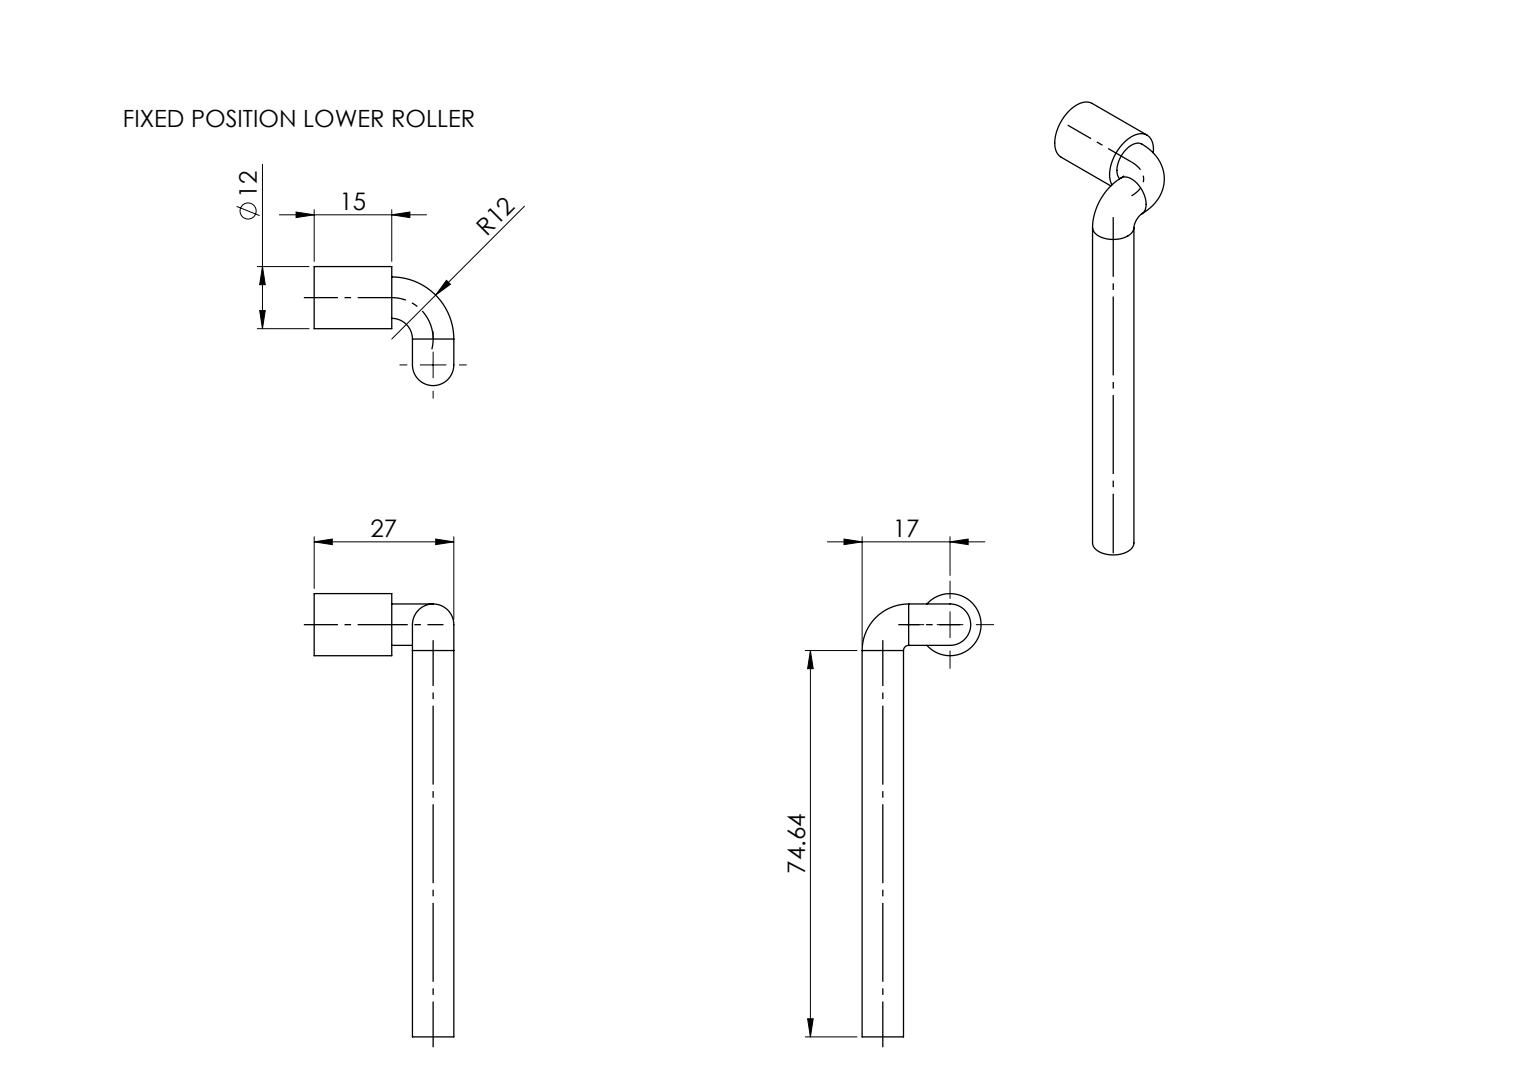
ISO-10303-21;
HEADER;
FILE_DESCRIPTION (('STEP AP214'),
    '1' );
FILE_NAME ('fixed position lower roller.step',
    '2026-10-03T20:08:58',
    ( '' ),
    ( '' ),
    'SwSTEP 2.0',
    'SolidWorks 2026',
    '' );
FILE_SCHEMA (( 'AUTOMOTIVE_DESIGN' ));
ENDSEC;

DATA;
#39=SHAPE_DEFINITION_REPRESENTATION ( #2484, #8378 ) ;
#44=PLANE ( 'NONE',  #3777 ) ;
#107=CIRCLE ( 'NONE', #5659, 4.000000000000001776 ) ;
#165=CARTESIAN_POINT ( 'NONE',  ( 14.00000000000000000, -30.00000000000000000, 0.000000000000000000 ) ) ;
#183=EDGE_CURVE ( 'NONE', #1508, #4176, #5201, .T. ) ;
#196=AXIS2_PLACEMENT_3D ( 'NONE', #1167, #8956, #10887 ) ;
#219=ORIENTED_EDGE ( 'NONE', *, *, #11430, .T. ) ;
#239=CIRCLE ( 'NONE', #9478, 4.000000000000001776 ) ;
#289=DIRECTION ( 'NONE',  ( 0.000000000000000000, 0.000000000000000000, 1.000000000000000000 ) ) ;
#309=CARTESIAN_POINT ( 'NONE',  ( 14.00000000000000000, 45.63999999999998636, -5.000000000000001776 ) ) ;
#315=DIRECTION ( 'NONE',  ( 0.000000000000000000, -1.000000000000000000, 0.000000000000000000 ) ) ;
#335=VERTEX_POINT ( 'NONE', #4396 ) ;
#383=CIRCLE ( 'NONE', #8612, 3.999999999999997335 ) ;
#411=DIRECTION ( 'NONE',  ( 1.000000000000000000, -0.000000000000000000, -0.000000000000000000 ) ) ;
#441=DIRECTION ( 'NONE',  ( 1.000000000000000000, 0.000000000000000000, 0.000000000000000000 ) ) ;
#461=( NAMED_UNIT ( * ) SI_UNIT ( $, .STERADIAN. ) SOLID_ANGLE_UNIT ( ) );
#467=DIRECTION ( 'NONE',  ( 0.000000000000000000, 0.000000000000000000, -1.000000000000000000 ) ) ;
#526=FILL_AREA_STYLE ('',( #12323 ) ) ;
#598=COLOUR_RGB ( '', 0.40784314, 0.44705882, 0.49803922) ;
#623=CIRCLE ( 'NONE', #8615, 4.000000000000001776 ) ;
#633=TOROIDAL_SURFACE ( 'NONE', #12373, 4.999999999999997335, 4.000000000000000000 ) ;
#644=AXIS2_PLACEMENT_3D ( 'NONE', #4663, #8717, #5810 ) ;
#663=EDGE_CURVE ( 'NONE', #8684, #9579, #239, .T. ) ;
#710=CIRCLE ( 'NONE', #1557, 12.00000000000000000 ) ;
#712=AXIS2_PLACEMENT_3D ( 'NONE', #10541, #1663, #1727 ) ;
#726=ADVANCED_FACE ( 'NONE', ( #8496 ), #11276, .T. ) ;
#750=DIRECTION ( 'NONE',  ( 0.000000000000000000, -1.000000000000000000, 0.000000000000000000 ) ) ;
#801=FACE_OUTER_BOUND ( 'NONE', #953, .T. ) ;
#853=CARTESIAN_POINT ( 'NONE',  ( 6.000000000000000000, 49.63999999999998636, -5.000000000000000888 ) ) ;
#868=ORIENTED_EDGE ( 'NONE', *, *, #10999, .F. ) ;
#953=EDGE_LOOP ( 'NONE', ( #2112, #9197, #11094, #219, #1705 ) ) ;
#990=ORIENTED_EDGE ( 'NONE', *, *, #11430, .F. ) ;
#1013=( GEOMETRIC_REPRESENTATION_CONTEXT ( 3 ) GLOBAL_UNCERTAINTY_ASSIGNED_CONTEXT ( ( #8516 ) ) GLOBAL_UNIT_ASSIGNED_CONTEXT ( ( #5432, #1437, #12211 ) ) REPRESENTATION_CONTEXT ( 'NONE', 'WORKASPACE' ) );
#1035=COLOUR_RGB ( '', 0.40784314, 0.44705882, 0.49803922) ;
#1075=EDGE_CURVE ( 'NONE', #9359, #4176, #10389, .T. ) ;
#1167=CARTESIAN_POINT ( 'NONE',  ( 6.000000000000000000, 49.63999999999998636, -13.00000000000000178 ) ) ;
#1182=VERTEX_POINT ( 'NONE', #6546 ) ;
#1304=CARTESIAN_POINT ( 'NONE',  ( 18.00000000000000355, 49.63999999999998636, -5.000000000000002665 ) ) ;
#1317=DIRECTION ( 'NONE',  ( 0.000000000000000000, -0.000000000000000000, -1.000000000000000000 ) ) ;
#1361=ORIENTED_EDGE ( 'NONE', *, *, #8700, .T. ) ;
#1370=EDGE_CURVE ( 'NONE', #1182, #3532, #383, .T. ) ;
#1431=PLANE ( 'NONE',  #6524 ) ;
#1437=( NAMED_UNIT ( * ) PLANE_ANGLE_UNIT ( ) SI_UNIT ( $, .RADIAN. ) );
#1456=DIRECTION ( 'NONE',  ( 0.000000000000000000, 0.000000000000000000, -1.000000000000000000 ) ) ;
#1467=CARTESIAN_POINT ( 'NONE',  ( -9.000000000000000000, 49.63999999999998636, -7.000000000000000888 ) ) ;
#1477=EDGE_CURVE ( 'NONE', #4665, #9359, #3885, .T. ) ;
#1508=VERTEX_POINT ( 'NONE', #12741 ) ;
#1527=CARTESIAN_POINT ( 'NONE',  ( 14.00000000000000000, -30.00000000000000000, 0.000000000000000000 ) ) ;
#1554=( NAMED_UNIT ( * ) PLANE_ANGLE_UNIT ( ) SI_UNIT ( $, .RADIAN. ) );
#1557=AXIS2_PLACEMENT_3D ( 'NONE', #2137, #6252, #4257 ) ;
#1576=DIRECTION ( 'NONE',  ( 0.000000000000000000, -1.000000000000000000, 0.000000000000000000 ) ) ;
#1583=DIRECTION ( 'NONE',  ( -1.000000000000000000, 0.000000000000000000, 0.000000000000000000 ) ) ;
#1615=SHAPE_REPRESENTATION_RELATIONSHIP ( 'NONE' , 'NONE' ,  #8378, #2668 ) ;
#1663=DIRECTION ( 'NONE',  ( 1.000000000000000000, -0.000000000000000000, -0.000000000000000000 ) ) ;
#1667=ADVANCED_FACE ( 'NONE', ( #7835 ), #4159, .T. ) ;
#1687=DIRECTION ( 'NONE',  ( 0.000000000000000000, 0.000000000000000000, 1.000000000000000000 ) ) ;
#1705=ORIENTED_EDGE ( 'NONE', *, *, #9638, .F. ) ;
#1721=DIRECTION ( 'NONE',  ( 0.000000000000000000, 0.000000000000000000, 1.000000000000000000 ) ) ;
#1727=DIRECTION ( 'NONE',  ( 0.000000000000000000, 0.000000000000000000, -1.000000000000000000 ) ) ;
#1775=ORIENTED_EDGE ( 'NONE', *, *, #8895, .T. ) ;
#1784=ORIENTED_EDGE ( 'NONE', *, *, #6220, .F. ) ;
#1797=ORIENTED_EDGE ( 'NONE', *, *, #2499, .F. ) ;
#1867=EDGE_LOOP ( 'NONE', ( #3480, #9604, #3827, #3918 ) ) ;
#2007=FACE_BOUND ( 'NONE', #4689, .T. ) ;
#2111=ORIENTED_EDGE ( 'NONE', *, *, #4710, .T. ) ;
#2112=ORIENTED_EDGE ( 'NONE', *, *, #6635, .F. ) ;
#2137=CARTESIAN_POINT ( 'NONE',  ( 6.000000000000000000, 49.63999999999998636, -5.000000000000000888 ) ) ;
#2180=ORIENTED_EDGE ( 'NONE', *, *, #9546, .F. ) ;
#2213=CARTESIAN_POINT ( 'NONE',  ( 6.000000000000000000, 49.63999999999998636, -13.00000000000000178 ) ) ;
#2355=SURFACE_STYLE_USAGE ( .BOTH. , #11170 ) ;
#2484=PRODUCT_DEFINITION_SHAPE ( 'NONE', 'NONE',  #5392 ) ;
#2492=EDGE_LOOP ( 'NONE', ( #5472, #2661, #6374, #990, #2581 ) ) ;
#2499=EDGE_CURVE ( 'NONE', #6983, #335, #11734, .T. ) ;
#2512=CARTESIAN_POINT ( 'NONE',  ( 14.00000000000000000, 49.63999999999998636, -5.000000000000001776 ) ) ;
#2540=CARTESIAN_POINT ( 'NONE',  ( -9.000000000000000000, 49.63999999999998636, -13.00000000000000178 ) ) ;
#2543=CARTESIAN_POINT ( 'NONE',  ( 14.00000000000000000, 61.31370849898475228, 3.999999999999997335 ) ) ;
#2565=ORIENTED_EDGE ( 'NONE', *, *, #663, .F. ) ;
#2581=ORIENTED_EDGE ( 'NONE', *, *, #4127, .T. ) ;
#2596=SURFACE_SIDE_STYLE ('',( #11353 ) ) ;
#2657=CARTESIAN_POINT ( 'NONE',  ( 14.00000000000000000, 49.63999999999998636, -5.000000000000001776 ) ) ;
#2661=ORIENTED_EDGE ( 'NONE', *, *, #6635, .T. ) ;
#2668=ADVANCED_BREP_SHAPE_REPRESENTATION ( '', ( #10172, #12422 ), #7225 ) ;
#2717=MECHANICAL_DESIGN_GEOMETRIC_PRESENTATION_REPRESENTATION('',(#4122),#5979);
#2801=AXIS2_PLACEMENT_3D ( 'NONE', #10218, #9264, #3434 ) ;
#2832=VERTEX_POINT ( 'NONE', #309 ) ;
#2874=DIRECTION ( 'NONE',  ( -0.000000000000000000, -1.000000000000000000, 0.000000000000000000 ) ) ;
#2906=APPLICATION_CONTEXT ( 'automotive_design' ) ;
#2926=ORIENTED_EDGE ( 'NONE', *, *, #1477, .F. ) ;
#3002=TOROIDAL_SURFACE ( 'NONE', #5451, 8.000000000000000000, 4.000000000000000000 ) ;
#3030=DIRECTION ( 'NONE',  ( 1.084202172485504434E-16, 0.000000000000000000, 1.000000000000000000 ) ) ;
#3084=DIRECTION ( 'NONE',  ( 0.000000000000000000, -1.000000000000000000, 0.000000000000000000 ) ) ;
#3123=ADVANCED_FACE ( 'NONE', ( #4941 ), #44, .T. ) ;
#3186=CYLINDRICAL_SURFACE ( 'NONE', #4205, 3.999999999999997335 ) ;
#3333=EDGE_LOOP ( 'NONE', ( #4773, #7781 ) ) ;
#3345=ORIENTED_EDGE ( 'NONE', *, *, #183, .F. ) ;
#3434=DIRECTION ( 'NONE',  ( 0.000000000000000000, 0.000000000000000000, 1.000000000000000000 ) ) ;
#3452=CARTESIAN_POINT ( 'NONE',  ( 14.00000000000000000, -30.00000000000000000, 0.000000000000000000 ) ) ;
#3480=ORIENTED_EDGE ( 'NONE', *, *, #7586, .T. ) ;
#3509=DIRECTION ( 'NONE',  ( 0.000000000000000000, -1.000000000000000000, 0.000000000000000000 ) ) ;
#3532=VERTEX_POINT ( 'NONE', #7691 ) ;
#3649=CARTESIAN_POINT ( 'NONE',  ( 14.00000000000000000, 61.31370849898475228, -3.999999999999997335 ) ) ;
#3777=AXIS2_PLACEMENT_3D ( 'NONE', #165, #3084, #1317 ) ;
#3801=CIRCLE ( 'NONE', #12246, 4.000000000000000000 ) ;
#3827=ORIENTED_EDGE ( 'NONE', *, *, #1370, .F. ) ;
#3856=PRODUCT_DEFINITION_FORMATION_WITH_SPECIFIED_SOURCE ( 'ANY', '', #11216, .NOT_KNOWN. ) ;
#3869=CARTESIAN_POINT ( 'NONE',  ( 6.000000000000000000, 49.63999999999998636, -5.000000000000000888 ) ) ;
#3885=CIRCLE ( 'NONE', #9832, 6.000000000000000000 ) ;
#3918=ORIENTED_EDGE ( 'NONE', *, *, #4710, .F. ) ;
#4087=ORIENTED_EDGE ( 'NONE', *, *, #7899, .F. ) ;
#4097=ORIENTED_EDGE ( 'NONE', *, *, #9546, .T. ) ;
#4122=STYLED_ITEM ( 'NONE', ( #5487 ), #2668 ) ;
#4127=EDGE_CURVE ( 'NONE', #2832, #8684, #4814, .T. ) ;
#4159=CYLINDRICAL_SURFACE ( 'NONE', #11300, 6.000000000000000000 ) ;
#4176=VERTEX_POINT ( 'NONE', #1467 ) ;
#4205=AXIS2_PLACEMENT_3D ( 'NONE', #9971, #11021, #9081 ) ;
#4257=DIRECTION ( 'NONE',  ( 0.000000000000000000, 0.000000000000000000, -1.000000000000000000 ) ) ;
#4314=AXIS2_PLACEMENT_3D ( 'NONE', #6303, #6240, #12180 ) ;
#4340=FILL_AREA_STYLE_COLOUR ( '', #598 ) ;
#4396=CARTESIAN_POINT ( 'NONE',  ( 6.000000000000000000, 49.63999999999998636, -17.00000000000000000 ) ) ;
#4457=( LENGTH_UNIT ( ) NAMED_UNIT ( * ) SI_UNIT ( .MILLI., .METRE. ) );
#4593=DIRECTION ( 'NONE',  ( -1.000000000000000000, 0.000000000000000000, 0.000000000000000000 ) ) ;
#4599=DIRECTION ( 'NONE',  ( 1.000000000000000000, 0.000000000000000000, 0.000000000000000000 ) ) ;
#4601=LINE ( 'NONE', #8514, #11819 ) ;
#4611=LINE ( 'NONE', #3649, #8149 ) ;
#4663=CARTESIAN_POINT ( 'NONE',  ( 14.00000000000000000, 44.64000000000000057, -5.000000000000000888 ) ) ;
#4665=VERTEX_POINT ( 'NONE', #12412 ) ;
#4689=EDGE_LOOP ( 'NONE', ( #1797, #11902 ) ) ;
#4710=EDGE_CURVE ( 'NONE', #9185, #1182, #4611, .T. ) ;
#4733=CIRCLE ( 'NONE', #4314, 6.000000000000000000 ) ;
#4735=DIRECTION ( 'NONE',  ( -1.000000000000000000, 0.000000000000000000, 0.000000000000000000 ) ) ;
#4773=ORIENTED_EDGE ( 'NONE', *, *, #10875, .T. ) ;
#4814=CIRCLE ( 'NONE', #10984, 4.000000000000001776 ) ;
#4941=FACE_OUTER_BOUND ( 'NONE', #6769, .T. ) ;
#4961=DIRECTION ( 'NONE',  ( 0.000000000000000000, 0.000000000000000000, -1.000000000000000000 ) ) ;
#5078=ADVANCED_FACE ( 'NONE', ( #6464 ), #1431, .F. ) ;
#5201=CIRCLE ( 'NONE', #7672, 6.000000000000000000 ) ;
#5365=DIRECTION ( 'NONE',  ( 0.000000000000000000, 0.000000000000000000, -1.000000000000000000 ) ) ;
#5382=CIRCLE ( 'NONE', #12189, 4.000000000000000000 ) ;
#5384=ORIENTED_EDGE ( 'NONE', *, *, #8895, .F. ) ;
#5392=PRODUCT_DEFINITION ( 'UNKNOWN', '', #3856, #11070 ) ;
#5429=CIRCLE ( 'NONE', #11614, 3.999999999999997335 ) ;
#5432=( LENGTH_UNIT ( ) NAMED_UNIT ( * ) SI_UNIT ( .MILLI., .METRE. ) );
#5451=AXIS2_PLACEMENT_3D ( 'NONE', #3869, #5728, #4961 ) ;
#5472=ORIENTED_EDGE ( 'NONE', *, *, #663, .T. ) ;
#5487=PRESENTATION_STYLE_ASSIGNMENT (( #10435 ) ) ;
#5503=FACE_OUTER_BOUND ( 'NONE', #2492, .T. ) ;
#5506=ORIENTED_EDGE ( 'NONE', *, *, #2499, .T. ) ;
#5566=FACE_OUTER_BOUND ( 'NONE', #9035, .T. ) ;
#5596=ORIENTED_EDGE ( 'NONE', *, *, #6633, .F. ) ;
#5659=AXIS2_PLACEMENT_3D ( 'NONE', #7893, #3030, #10920 ) ;
#5706=ORIENTED_EDGE ( 'NONE', *, *, #8700, .F. ) ;
#5707=CARTESIAN_POINT ( 'NONE',  ( 0.000000000000000000, 0.000000000000000000, 0.000000000000000000 ) ) ;
#5728=DIRECTION ( 'NONE',  ( -0.000000000000000000, -1.000000000000000000, 0.000000000000000000 ) ) ;
#5754=AXIS2_PLACEMENT_3D ( 'NONE', #6221, #10326, #1456 ) ;
#5774=DIRECTION ( 'NONE',  ( -0.000000000000000000, -1.000000000000000000, 0.000000000000000000 ) ) ;
#5810=DIRECTION ( 'NONE',  ( 0.000000000000000000, 0.000000000000000000, -1.000000000000000000 ) ) ;
#5825=DIRECTION ( 'NONE',  ( 0.000000000000000000, 0.000000000000000000, -1.000000000000000000 ) ) ;
#5953=ORIENTED_EDGE ( 'NONE', *, *, #1477, .T. ) ;
#5979=( GEOMETRIC_REPRESENTATION_CONTEXT ( 3 ) GLOBAL_UNCERTAINTY_ASSIGNED_CONTEXT ( ( #10346 ) ) GLOBAL_UNIT_ASSIGNED_CONTEXT ( ( #11284, #8444, #461 ) ) REPRESENTATION_CONTEXT ( 'NONE', 'WORKASPACE' ) );
#6059=FACE_OUTER_BOUND ( 'NONE', #12004, .T. ) ;
#6106=ORIENTED_EDGE ( 'NONE', *, *, #11647, .T. ) ;
#6130=DIRECTION ( 'NONE',  ( 0.000000000000000000, 0.000000000000000000, 1.000000000000000000 ) ) ;
#6140=DIRECTION ( 'NONE',  ( 0.000000000000000000, -1.000000000000000000, 0.000000000000000000 ) ) ;
#6173=AXIS2_PLACEMENT_3D ( 'NONE', #9380, #8432, #11275 ) ;
#6195=CIRCLE ( 'NONE', #644, 0.9999999999999974465 ) ;
#6220=EDGE_CURVE ( 'NONE', #11818, #3532, #12396, .T. ) ;
#6221=CARTESIAN_POINT ( 'NONE',  ( 14.00000000000000000, 61.31370849898475228, 0.000000000000000000 ) ) ;
#6240=DIRECTION ( 'NONE',  ( -1.000000000000000000, 0.000000000000000000, 0.000000000000000000 ) ) ;
#6252=DIRECTION ( 'NONE',  ( -0.000000000000000000, -1.000000000000000000, 0.000000000000000000 ) ) ;
#6288=FACE_OUTER_BOUND ( 'NONE', #1867, .T. ) ;
#6303=CARTESIAN_POINT ( 'NONE',  ( 6.000000000000000000, 49.63999999999998636, -13.00000000000000178 ) ) ;
#6367=STYLED_ITEM ( 'NONE', ( #11365 ), #10172 ) ;
#6374=ORIENTED_EDGE ( 'NONE', *, *, #7586, .F. ) ;
#6398=CARTESIAN_POINT ( 'NONE',  ( -9.000000000000000000, 49.63999999999998636, -13.00000000000000178 ) ) ;
#6423=ORIENTED_EDGE ( 'NONE', *, *, #1370, .T. ) ;
#6425=CARTESIAN_POINT ( 'NONE',  ( -9.000000000000000000, 49.63999999999998636, -13.00000000000000178 ) ) ;
#6428=DIRECTION ( 'NONE',  ( 1.000000000000000000, 0.000000000000000000, 0.000000000000000000 ) ) ;
#6464=FACE_OUTER_BOUND ( 'NONE', #3333, .T. ) ;
#6501=DIRECTION ( 'NONE',  ( 1.084202172485504434E-16, 0.000000000000000000, 1.000000000000000000 ) ) ;
#6524=AXIS2_PLACEMENT_3D ( 'NONE', #6398, #10233, #467 ) ;
#6546=CARTESIAN_POINT ( 'NONE',  ( 14.00000000000000000, -30.00000000000000000, -3.999999999999997335 ) ) ;
#6598=AXIS2_PLACEMENT_3D ( 'NONE', #6425, #1583, #12053 ) ;
#6633=EDGE_CURVE ( 'NONE', #6983, #8089, #3801, .T. ) ;
#6635=EDGE_CURVE ( 'NONE', #9579, #11818, #11832, .T. ) ;
#6682=DIRECTION ( 'NONE',  ( 1.084202172485504434E-16, 0.000000000000000000, 1.000000000000000000 ) ) ;
#6696=CARTESIAN_POINT ( 'NONE',  ( 6.000000000000000000, 49.63999999999998636, -5.000000000000000888 ) ) ;
#6698=ORIENTED_EDGE ( 'NONE', *, *, #10875, .F. ) ;
#6767=CARTESIAN_POINT ( 'NONE',  ( 10.00000000000000000, 49.63999999999998636, -5.000000000000000888 ) ) ;
#6769=EDGE_LOOP ( 'NONE', ( #6423, #1361 ) ) ;
#6846=EDGE_CURVE ( 'NONE', #8089, #2832, #107, .T. ) ;
#6870=EDGE_LOOP ( 'NONE', ( #5384, #5953, #11441, #3345 ) ) ;
#6941=VECTOR ( 'NONE', #12458, 1000.000000000000000 ) ;
#6983=VERTEX_POINT ( 'NONE', #12097 ) ;
#7125=DIRECTION ( 'NONE',  ( -1.000000000000000000, 0.000000000000000000, 0.000000000000000000 ) ) ;
#7225=( GEOMETRIC_REPRESENTATION_CONTEXT ( 3 ) GLOBAL_UNCERTAINTY_ASSIGNED_CONTEXT ( ( #9438 ) ) GLOBAL_UNIT_ASSIGNED_CONTEXT ( ( #4457, #1554, #9150 ) ) REPRESENTATION_CONTEXT ( 'NONE', 'WORKASPACE' ) );
#7249=AXIS2_PLACEMENT_3D ( 'NONE', #853, #2874, #11681 ) ;
#7371=SURFACE_STYLE_FILL_AREA ( #10239 ) ;
#7392=DIRECTION ( 'NONE',  ( 0.000000000000000000, 0.000000000000000000, 1.000000000000000000 ) ) ;
#7434=DIRECTION ( 'NONE',  ( -1.000000000000000000, 0.000000000000000000, 0.000000000000000000 ) ) ;
#7586=EDGE_CURVE ( 'NONE', #9185, #11818, #8122, .T. ) ;
#7664=CLOSED_SHELL ( 'NONE', ( #11318, #8093, #726, #9848, #3123, #7850, #9969, #11541, #1667, #10336, #5078 ) ) ;
#7672=AXIS2_PLACEMENT_3D ( 'NONE', #2540, #4593, #1687 ) ;
#7691=CARTESIAN_POINT ( 'NONE',  ( 14.00000000000000000, -30.00000000000000000, 3.999999999999997335 ) ) ;
#7781=ORIENTED_EDGE ( 'NONE', *, *, #183, .T. ) ;
#7829=DIRECTION ( 'NONE',  ( 1.000000000000000000, 0.000000000000000000, -2.168404344971007882E-16 ) ) ;
#7835=FACE_OUTER_BOUND ( 'NONE', #6870, .T. ) ;
#7850=ADVANCED_FACE ( 'NONE', ( #6059 ), #3186, .T. ) ;
#7869=PLANE ( 'NONE',  #196 ) ;
#7893=CARTESIAN_POINT ( 'NONE',  ( 14.00000000000000000, 49.63999999999998636, -5.000000000000001776 ) ) ;
#7899=EDGE_CURVE ( 'NONE', #335, #8684, #710, .T. ) ;
#8067=EDGE_LOOP ( 'NONE', ( #2180, #2926 ) ) ;
#8072=PRODUCT_CONTEXT ( 'NONE', #12271, 'mechanical' ) ;
#8089=VERTEX_POINT ( 'NONE', #6767 ) ;
#8093=ADVANCED_FACE ( 'NONE', ( #8695 ), #3002, .T. ) ;
#8101=CARTESIAN_POINT ( 'NONE',  ( 14.00000000000000000, 53.63999999999999346, -5.000000000000001776 ) ) ;
#8122=CIRCLE ( 'NONE', #12055, 4.000000000000001776 ) ;
#8149=VECTOR ( 'NONE', #1576, 1000.000000000000000 ) ;
#8174=CARTESIAN_POINT ( 'NONE',  ( 14.00000000000000000, 44.64000000000000057, -6.938893903907228378E-15 ) ) ;
#8253=CARTESIAN_POINT ( 'NONE',  ( 14.00000000000000000, 44.64000000000000057, -4.000000000000007105 ) ) ;
#8265=TOROIDAL_SURFACE ( 'NONE', #7249, 8.000000000000000000, 4.000000000000000000 ) ;
#8378=SHAPE_REPRESENTATION ( 'fixed position lower roller', ( #12422 ), #7225 ) ;
#8432=DIRECTION ( 'NONE',  ( 1.000000000000000000, -0.000000000000000000, -0.000000000000000000 ) ) ;
#8444=( NAMED_UNIT ( * ) PLANE_ANGLE_UNIT ( ) SI_UNIT ( $, .RADIAN. ) );
#8496=FACE_OUTER_BOUND ( 'NONE', #12428, .T. ) ;
#8499=CARTESIAN_POINT ( 'NONE',  ( 6.000000000000000000, 49.63999999999998636, -7.000000000000000888 ) ) ;
#8514=CARTESIAN_POINT ( 'NONE',  ( 6.000000000000000000, 49.63999999999998636, -19.00000000000000355 ) ) ;
#8516=UNCERTAINTY_MEASURE_WITH_UNIT (LENGTH_MEASURE( 1.000000000000000082E-05 ), #5432, 'distance_accuracy_value', 'NONE');
#8591=CARTESIAN_POINT ( 'NONE',  ( 6.000000000000000000, 49.63999999999998636, -7.000000000000000888 ) ) ;
#8612=AXIS2_PLACEMENT_3D ( 'NONE', #1527, #750, #10598 ) ;
#8615=AXIS2_PLACEMENT_3D ( 'NONE', #9610, #6682, #7829 ) ;
#8629=VECTOR ( 'NONE', #4735, 1000.000000000000000 ) ;
#8684=VERTEX_POINT ( 'NONE', #1304 ) ;
#8695=FACE_OUTER_BOUND ( 'NONE', #11687, .T. ) ;
#8700=EDGE_CURVE ( 'NONE', #3532, #1182, #5429, .T. ) ;
#8717=DIRECTION ( 'NONE',  ( 1.000000000000000000, -0.000000000000000000, -0.000000000000000000 ) ) ;
#8857=ORIENTED_EDGE ( 'NONE', *, *, #4127, .F. ) ;
#8895=EDGE_CURVE ( 'NONE', #4665, #1508, #4601, .T. ) ;
#8956=DIRECTION ( 'NONE',  ( -1.000000000000000000, 0.000000000000000000, 0.000000000000000000 ) ) ;
#9035=EDGE_LOOP ( 'NONE', ( #4087, #6106, #9609, #868, #2565 ) ) ;
#9045=CARTESIAN_POINT ( 'NONE',  ( 6.000000000000000000, 49.63999999999998636, -13.00000000000000178 ) ) ;
#9081=DIRECTION ( 'NONE',  ( 0.000000000000000000, 0.000000000000000000, -1.000000000000000000 ) ) ;
#9150=( NAMED_UNIT ( * ) SI_UNIT ( $, .STERADIAN. ) SOLID_ANGLE_UNIT ( ) );
#9185=VERTEX_POINT ( 'NONE', #8253 ) ;
#9197=ORIENTED_EDGE ( 'NONE', *, *, #10999, .T. ) ;
#9264=DIRECTION ( 'NONE',  ( -1.000000000000000000, 0.000000000000000000, 0.000000000000000000 ) ) ;
#9268=TOROIDAL_SURFACE ( 'NONE', #12182, 4.999999999999997335, 4.000000000000000000 ) ;
#9359=VERTEX_POINT ( 'NONE', #8499 ) ;
#9380=CARTESIAN_POINT ( 'NONE',  ( 6.000000000000000000, 49.63999999999998636, -13.00000000000000178 ) ) ;
#9404=CARTESIAN_POINT ( 'NONE',  ( 14.00000000000000000, 44.64000000000000057, -5.000000000000000888 ) ) ;
#9437=CIRCLE ( 'NONE', #11721, 4.000000000000001776 ) ;
#9438=UNCERTAINTY_MEASURE_WITH_UNIT (LENGTH_MEASURE( 1.000000000000000082E-05 ), #4457, 'distance_accuracy_value', 'NONE');
#9467=CARTESIAN_POINT ( 'NONE',  ( 14.00000000000000000, 44.64000000000000057, -6.938893903907228378E-15 ) ) ;
#9478=AXIS2_PLACEMENT_3D ( 'NONE', #2657, #11344, #10426 ) ;
#9546=EDGE_CURVE ( 'NONE', #9359, #4665, #4733, .T. ) ;
#9563=DIRECTION ( 'NONE',  ( 0.000000000000000000, 0.000000000000000000, -1.000000000000000000 ) ) ;
#9579=VERTEX_POINT ( 'NONE', #8101 ) ;
#9604=ORIENTED_EDGE ( 'NONE', *, *, #6220, .T. ) ;
#9609=ORIENTED_EDGE ( 'NONE', *, *, #6633, .T. ) ;
#9610=CARTESIAN_POINT ( 'NONE',  ( 14.00000000000000000, 49.63999999999998636, -5.000000000000001776 ) ) ;
#9619=CARTESIAN_POINT ( 'NONE',  ( 6.000000000000000000, 49.63999999999998636, -13.00000000000000178 ) ) ;
#9638=EDGE_CURVE ( 'NONE', #11818, #9185, #9437, .T. ) ;
#9832=AXIS2_PLACEMENT_3D ( 'NONE', #9619, #12617, #1721 ) ;
#9848=ADVANCED_FACE ( 'NONE', ( #6288 ), #10261, .T. ) ;
#9969=ADVANCED_FACE ( 'NONE', ( #801 ), #633, .T. ) ;
#9971=CARTESIAN_POINT ( 'NONE',  ( 14.00000000000000000, 61.31370849898475228, 0.000000000000000000 ) ) ;
#9975=DIRECTION ( 'NONE',  ( 1.000000000000000000, -0.000000000000000000, -0.000000000000000000 ) ) ;
#10172=MANIFOLD_SOLID_BREP ( 'Boss-Extrude2', #7664 ) ;
#10218=CARTESIAN_POINT ( 'NONE',  ( 6.000000000000000000, 49.63999999999998636, -13.00000000000000178 ) ) ;
#10233=DIRECTION ( 'NONE',  ( 1.000000000000000000, 0.000000000000000000, 0.000000000000000000 ) ) ;
#10239=FILL_AREA_STYLE ('',( #4340 ) ) ;
#10243=DIRECTION ( 'NONE',  ( 0.000000000000000000, 0.000000000000000000, -1.000000000000000000 ) ) ;
#10261=CYLINDRICAL_SURFACE ( 'NONE', #5754, 3.999999999999997335 ) ;
#10326=DIRECTION ( 'NONE',  ( 0.000000000000000000, -1.000000000000000000, 0.000000000000000000 ) ) ;
#10336=ADVANCED_FACE ( 'NONE', ( #2007, #10757 ), #7869, .F. ) ;
#10346=UNCERTAINTY_MEASURE_WITH_UNIT (LENGTH_MEASURE( 1.000000000000000082E-05 ), #11284, 'distance_accuracy_value', 'NONE');
#10389=LINE ( 'NONE', #8591, #8629 ) ;
#10426=DIRECTION ( 'NONE',  ( 1.000000000000000000, 0.000000000000000000, -2.168404344971007882E-16 ) ) ;
#10435=SURFACE_STYLE_USAGE ( .BOTH. , #2596 ) ;
#10541=CARTESIAN_POINT ( 'NONE',  ( 14.00000000000000000, 44.64000000000000057, -5.000000000000000888 ) ) ;
#10598=DIRECTION ( 'NONE',  ( 0.000000000000000000, 0.000000000000000000, -1.000000000000000000 ) ) ;
#10757=FACE_OUTER_BOUND ( 'NONE', #8067, .T. ) ;
#10875=EDGE_CURVE ( 'NONE', #4176, #1508, #11113, .T. ) ;
#10887=DIRECTION ( 'NONE',  ( 0.000000000000000000, 0.000000000000000000, 1.000000000000000000 ) ) ;
#10920=DIRECTION ( 'NONE',  ( 1.000000000000000000, 0.000000000000000000, -2.168404344971007882E-16 ) ) ;
#10984=AXIS2_PLACEMENT_3D ( 'NONE', #2512, #6501, #12370 ) ;
#10999=EDGE_CURVE ( 'NONE', #9579, #8089, #623, .T. ) ;
#11021=DIRECTION ( 'NONE',  ( 0.000000000000000000, -1.000000000000000000, 0.000000000000000000 ) ) ;
#11070=PRODUCT_DEFINITION_CONTEXT ( 'detailed design', #2906, 'design' ) ;
#11094=ORIENTED_EDGE ( 'NONE', *, *, #6846, .T. ) ;
#11113=CIRCLE ( 'NONE', #6598, 6.000000000000000000 ) ;
#11170=SURFACE_SIDE_STYLE ('',( #7371 ) ) ;
#11191=ORIENTED_EDGE ( 'NONE', *, *, #6846, .F. ) ;
#11216=PRODUCT ( 'fixed position lower roller', 'fixed position lower roller', '', ( #8072 ) ) ;
#11275=DIRECTION ( 'NONE',  ( 0.000000000000000000, 0.000000000000000000, 1.000000000000000000 ) ) ;
#11276=CYLINDRICAL_SURFACE ( 'NONE', #2801, 6.000000000000000000 ) ;
#11284=( LENGTH_UNIT ( ) NAMED_UNIT ( * ) SI_UNIT ( .MILLI., .METRE. ) );
#11300=AXIS2_PLACEMENT_3D ( 'NONE', #9045, #7125, #289 ) ;
#11318=ADVANCED_FACE ( 'NONE', ( #5503 ), #9268, .T. ) ;
#11344=DIRECTION ( 'NONE',  ( 1.084202172485504434E-16, 0.000000000000000000, 1.000000000000000000 ) ) ;
#11353=SURFACE_STYLE_FILL_AREA ( #526 ) ;
#11365=PRESENTATION_STYLE_ASSIGNMENT (( #2355 ) ) ;
#11430=EDGE_CURVE ( 'NONE', #2832, #9185, #6195, .T. ) ;
#11441=ORIENTED_EDGE ( 'NONE', *, *, #1075, .T. ) ;
#11509=DIRECTION ( 'NONE',  ( 1.000000000000000000, -0.000000000000000000, -0.000000000000000000 ) ) ;
#11541=ADVANCED_FACE ( 'NONE', ( #5566 ), #8265, .T. ) ;
#11604=CARTESIAN_POINT ( 'NONE',  ( 14.00000000000000000, 44.64000000000000057, 3.999999999999993339 ) ) ;
#11614=AXIS2_PLACEMENT_3D ( 'NONE', #3452, #6140, #5365 ) ;
#11630=CARTESIAN_POINT ( 'NONE',  ( 14.00000000000000000, 44.64000000000000057, -5.000000000000000888 ) ) ;
#11647=EDGE_CURVE ( 'NONE', #335, #6983, #5382, .T. ) ;
#11681=DIRECTION ( 'NONE',  ( 0.000000000000000000, 0.000000000000000000, -1.000000000000000000 ) ) ;
#11687=EDGE_LOOP ( 'NONE', ( #5506, #12108, #8857, #11191, #5596 ) ) ;
#11721=AXIS2_PLACEMENT_3D ( 'NONE', #8174, #315, #441 ) ;
#11734=CIRCLE ( 'NONE', #6173, 4.000000000000000000 ) ;
#11818=VERTEX_POINT ( 'NONE', #11604 ) ;
#11819=VECTOR ( 'NONE', #7434, 1000.000000000000000 ) ;
#11832=CIRCLE ( 'NONE', #712, 8.999999999999998224 ) ;
#11887=ORIENTED_EDGE ( 'NONE', *, *, #9638, .T. ) ;
#11902=ORIENTED_EDGE ( 'NONE', *, *, #11647, .F. ) ;
#12004=EDGE_LOOP ( 'NONE', ( #1784, #11887, #2111, #5706 ) ) ;
#12053=DIRECTION ( 'NONE',  ( 0.000000000000000000, 0.000000000000000000, 1.000000000000000000 ) ) ;
#12055=AXIS2_PLACEMENT_3D ( 'NONE', #9467, #3509, #4599 ) ;
#12097=CARTESIAN_POINT ( 'NONE',  ( 6.000000000000000000, 49.63999999999998636, -9.000000000000001776 ) ) ;
#12108=ORIENTED_EDGE ( 'NONE', *, *, #7899, .T. ) ;
#12180=DIRECTION ( 'NONE',  ( 0.000000000000000000, 0.000000000000000000, 1.000000000000000000 ) ) ;
#12182=AXIS2_PLACEMENT_3D ( 'NONE', #9404, #411, #10243 ) ;
#12189=AXIS2_PLACEMENT_3D ( 'NONE', #2213, #9975, #6130 ) ;
#12211=( NAMED_UNIT ( * ) SI_UNIT ( $, .STERADIAN. ) SOLID_ANGLE_UNIT ( ) );
#12246=AXIS2_PLACEMENT_3D ( 'NONE', #6696, #5774, #9563 ) ;
#12271=APPLICATION_CONTEXT ( 'automotive_design' ) ;
#12323=FILL_AREA_STYLE_COLOUR ( '', #1035 ) ;
#12348=MECHANICAL_DESIGN_GEOMETRIC_PRESENTATION_REPRESENTATION('',(#6367),#1013);
#12370=DIRECTION ( 'NONE',  ( 1.000000000000000000, 0.000000000000000000, -2.168404344971007882E-16 ) ) ;
#12373=AXIS2_PLACEMENT_3D ( 'NONE', #11630, #11509, #5825 ) ;
#12387=ORIENTED_EDGE ( 'NONE', *, *, #1075, .F. ) ;
#12396=LINE ( 'NONE', #2543, #6941 ) ;
#12412=CARTESIAN_POINT ( 'NONE',  ( 6.000000000000000000, 49.63999999999998636, -19.00000000000000355 ) ) ;
#12422=AXIS2_PLACEMENT_3D ( 'NONE', #5707, #7392, #6428 ) ;
#12428=EDGE_LOOP ( 'NONE', ( #4097, #1775, #6698, #12387 ) ) ;
#12458=DIRECTION ( 'NONE',  ( 0.000000000000000000, -1.000000000000000000, 0.000000000000000000 ) ) ;
#12617=DIRECTION ( 'NONE',  ( -1.000000000000000000, 0.000000000000000000, 0.000000000000000000 ) ) ;
#12741=CARTESIAN_POINT ( 'NONE',  ( -9.000000000000000000, 49.63999999999998636, -19.00000000000000355 ) ) ;
ENDSEC;
END-ISO-10303-21;
